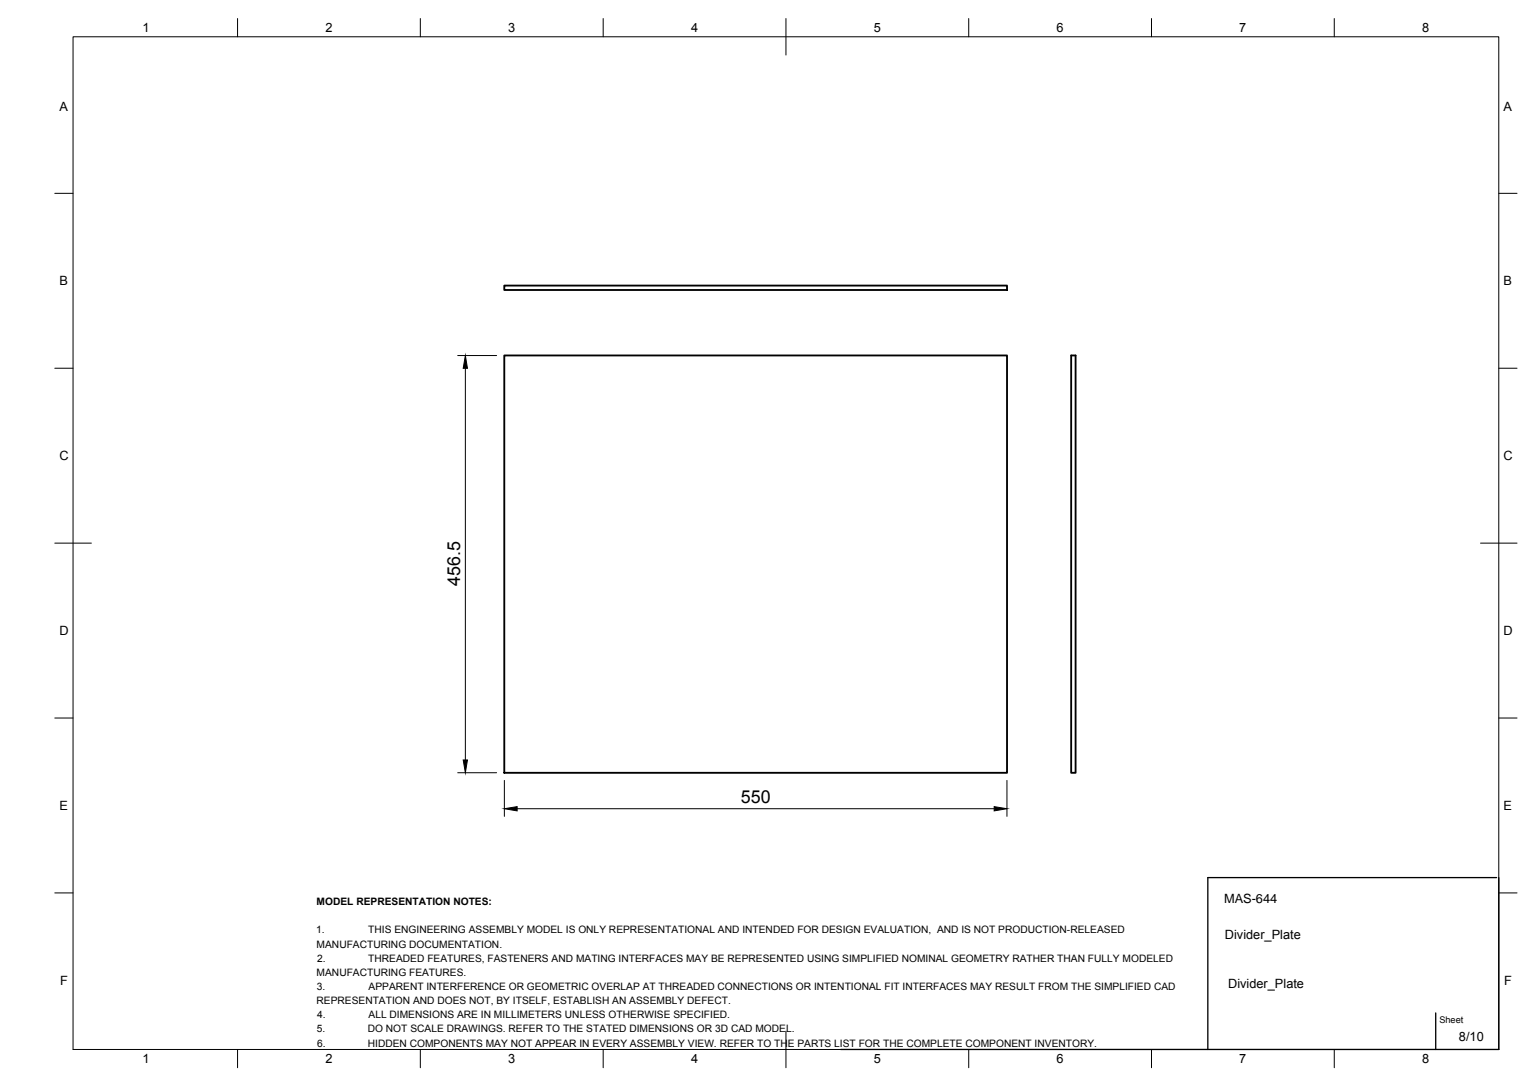
ISO-10303-21;
HEADER;
FILE_DESCRIPTION((''),'2;1');
FILE_NAME('Divider_Plate.step','2026-10-09T11:38:21-07:00',(''),(''),'','','');
FILE_SCHEMA (('AUTOMOTIVE_DESIGN { 1 0 10303 214 3 1 1 }'));
ENDSEC;
DATA;
#10=MECHANICAL_DESIGN_GEOMETRIC_PRESENTATION_REPRESENTATION('',(#64),#3619);
#48=SHAPE_REPRESENTATION_RELATIONSHIP('SRR','None',#3656,#56) ;
#56=ADVANCED_BREP_SHAPE_REPRESENTATION('',(#72),#3616) ;
#64=STYLED_ITEM('',(#3700),#72) ;
#72=MANIFOLD_SOLID_BREP('Body1',#2088) ;
#191=PLANE('',#2365) ;
#192=PLANE('',#2366) ;
#193=PLANE('',#2367) ;
#194=PLANE('',#2368) ;
#195=PLANE('',#2369) ;
#196=PLANE('',#2370) ;
#295=FACE_OUTER_BOUND('',#485,.T.) ;
#296=FACE_OUTER_BOUND('',#486,.T.) ;
#297=FACE_OUTER_BOUND('',#487,.T.) ;
#298=FACE_OUTER_BOUND('',#488,.T.) ;
#299=FACE_OUTER_BOUND('',#489,.T.) ;
#300=FACE_OUTER_BOUND('',#490,.T.) ;
#485=EDGE_LOOP('',(#1819,#1820,#1821,#1822)) ;
#486=EDGE_LOOP('',(#1823,#1824,#1825,#1826)) ;
#487=EDGE_LOOP('',(#1827,#1828,#1829,#1830)) ;
#488=EDGE_LOOP('',(#1831,#1832,#1833,#1834)) ;
#489=EDGE_LOOP('',(#1835,#1836,#1837,#1838)) ;
#490=EDGE_LOOP('',(#1839,#1840,#1841,#1842)) ;
#631=LINE('',#3483,#795) ;
#632=LINE('',#3485,#796) ;
#633=LINE('',#3487,#797) ;
#634=LINE('',#3488,#798) ;
#635=LINE('',#3491,#799) ;
#636=LINE('',#3493,#800) ;
#637=LINE('',#3494,#801) ;
#638=LINE('',#3497,#802) ;
#639=LINE('',#3499,#803) ;
#640=LINE('',#3500,#804) ;
#641=LINE('',#3502,#805) ;
#642=LINE('',#3503,#806) ;
#795=VECTOR('',#2901,1000.) ;
#796=VECTOR('',#2902,1000.) ;
#797=VECTOR('',#2903,1000.) ;
#798=VECTOR('',#2904,1000.) ;
#799=VECTOR('',#2907,1000.) ;
#800=VECTOR('',#2908,1000.) ;
#801=VECTOR('',#2909,1000.) ;
#802=VECTOR('',#2912,1000.) ;
#803=VECTOR('',#2913,1000.) ;
#804=VECTOR('',#2914,1000.) ;
#805=VECTOR('',#2917,1000.) ;
#806=VECTOR('',#2918,1000.) ;
#1087=VERTEX_POINT('',#3481) ;
#1088=VERTEX_POINT('',#3482) ;
#1089=VERTEX_POINT('',#3484) ;
#1090=VERTEX_POINT('',#3486) ;
#1091=VERTEX_POINT('',#3490) ;
#1092=VERTEX_POINT('',#3492) ;
#1093=VERTEX_POINT('',#3496) ;
#1094=VERTEX_POINT('',#3498) ;
#1335=EDGE_CURVE('',#1087,#1088,#631,.T.) ;
#1336=EDGE_CURVE('',#1089,#1087,#632,.T.) ;
#1337=EDGE_CURVE('',#1089,#1090,#633,.T.) ;
#1338=EDGE_CURVE('',#1090,#1088,#634,.T.) ;
#1339=EDGE_CURVE('',#1091,#1087,#635,.T.) ;
#1340=EDGE_CURVE('',#1092,#1091,#636,.T.) ;
#1341=EDGE_CURVE('',#1092,#1089,#637,.T.) ;
#1342=EDGE_CURVE('',#1093,#1091,#638,.T.) ;
#1343=EDGE_CURVE('',#1094,#1093,#639,.T.) ;
#1344=EDGE_CURVE('',#1094,#1092,#640,.T.) ;
#1345=EDGE_CURVE('',#1088,#1093,#641,.T.) ;
#1346=EDGE_CURVE('',#1090,#1094,#642,.T.) ;
#1819=ORIENTED_EDGE('',*,*,#1335,.F.) ;
#1820=ORIENTED_EDGE('',*,*,#1336,.F.) ;
#1821=ORIENTED_EDGE('',*,*,#1337,.T.) ;
#1822=ORIENTED_EDGE('',*,*,#1338,.T.) ;
#1823=ORIENTED_EDGE('',*,*,#1339,.F.) ;
#1824=ORIENTED_EDGE('',*,*,#1340,.F.) ;
#1825=ORIENTED_EDGE('',*,*,#1341,.T.) ;
#1826=ORIENTED_EDGE('',*,*,#1336,.T.) ;
#1827=ORIENTED_EDGE('',*,*,#1342,.F.) ;
#1828=ORIENTED_EDGE('',*,*,#1343,.F.) ;
#1829=ORIENTED_EDGE('',*,*,#1344,.T.) ;
#1830=ORIENTED_EDGE('',*,*,#1340,.T.) ;
#1831=ORIENTED_EDGE('',*,*,#1345,.F.) ;
#1832=ORIENTED_EDGE('',*,*,#1338,.F.) ;
#1833=ORIENTED_EDGE('',*,*,#1346,.T.) ;
#1834=ORIENTED_EDGE('',*,*,#1343,.T.) ;
#1835=ORIENTED_EDGE('',*,*,#1337,.F.) ;
#1836=ORIENTED_EDGE('',*,*,#1341,.F.) ;
#1837=ORIENTED_EDGE('',*,*,#1344,.F.) ;
#1838=ORIENTED_EDGE('',*,*,#1346,.F.) ;
#1839=ORIENTED_EDGE('',*,*,#1335,.T.) ;
#1840=ORIENTED_EDGE('',*,*,#1345,.T.) ;
#1841=ORIENTED_EDGE('',*,*,#1342,.T.) ;
#1842=ORIENTED_EDGE('',*,*,#1339,.T.) ;
#2057=ADVANCED_FACE('',(#295),#191,.T.) ;
#2058=ADVANCED_FACE('',(#296),#192,.T.) ;
#2059=ADVANCED_FACE('',(#297),#193,.T.) ;
#2060=ADVANCED_FACE('',(#298),#194,.T.) ;
#2061=ADVANCED_FACE('',(#299),#195,.F.) ;
#2062=ADVANCED_FACE('',(#300),#196,.T.) ;
#2088=CLOSED_SHELL('',(#2057,#2058,#2059,#2060,#2061,#2062)) ;
#2364=AXIS2_PLACEMENT_3D('',#3479,#2897,#2898) ;
#2365=AXIS2_PLACEMENT_3D('',#3480,#2899,#2900) ;
#2366=AXIS2_PLACEMENT_3D('',#3489,#2905,#2906) ;
#2367=AXIS2_PLACEMENT_3D('',#3495,#2910,#2911) ;
#2368=AXIS2_PLACEMENT_3D('',#3501,#2915,#2916) ;
#2369=AXIS2_PLACEMENT_3D('',#3504,#2919,#2920) ;
#2370=AXIS2_PLACEMENT_3D('',#3505,#2921,#2922) ;
#2897=DIRECTION('axis',(0.,0.,1.)) ;
#2898=DIRECTION('refdir',(1.,0.,0.)) ;
#2899=DIRECTION('center_axis',(3.11423403168202E-19,-2.44394566430984E-20,
1.)) ;
#2900=DIRECTION('ref_axis',(1.,-1.80411241501588E-16,-3.11423403168202E-19)) ;
#2901=DIRECTION('',(1.80411241501588E-16,1.,2.44394566430984E-20)) ;
#2902=DIRECTION('',(-1.,1.80411241501588E-16,3.11423403168202E-19)) ;
#2903=DIRECTION('',(1.80411241501588E-16,1.,2.44394566430984E-20)) ;
#2904=DIRECTION('',(-1.,1.80411241501588E-16,3.11423403168202E-19)) ;
#2905=DIRECTION('center_axis',(-1.80411241501588E-16,-1.,-2.44394566430983E-20)) ;
#2906=DIRECTION('ref_axis',(1.,-1.80411241501588E-16,-3.11423403168202E-19)) ;
#2907=DIRECTION('',(3.11423403168202E-19,-2.44394566430984E-20,1.)) ;
#2908=DIRECTION('',(-1.,1.80411241501588E-16,3.11423403168202E-19)) ;
#2909=DIRECTION('',(3.11423403168202E-19,-2.44394566430984E-20,1.)) ;
#2910=DIRECTION('center_axis',(-3.11423403168238E-19,-2.01834292293385E-16,
-1.)) ;
#2911=DIRECTION('ref_axis',(-1.80411241501588E-16,-1.,2.01834292293385E-16)) ;
#2912=DIRECTION('',(-1.80411241501588E-16,-1.,2.01834292293385E-16)) ;
#2913=DIRECTION('',(-1.,1.80411241501588E-16,3.11423403168202E-19)) ;
#2914=DIRECTION('',(-1.80411241501588E-16,-1.,2.01834292293385E-16)) ;
#2915=DIRECTION('center_axis',(1.80411241501588E-16,1.,2.44394566430983E-20)) ;
#2916=DIRECTION('ref_axis',(-1.,1.80411241501588E-16,3.11423403168202E-19)) ;
#2917=DIRECTION('',(-3.11423403168202E-19,2.44394566430984E-20,-1.)) ;
#2918=DIRECTION('',(-3.11423403168202E-19,2.44394566430984E-20,-1.)) ;
#2919=DIRECTION('center_axis',(-1.,1.80411241501588E-16,3.11423403168202E-19)) ;
#2920=DIRECTION('ref_axis',(3.11423403168202E-19,-2.44394566430984E-20,
1.)) ;
#2921=DIRECTION('center_axis',(-1.,1.80411241501588E-16,3.11423403168202E-19)) ;
#2922=DIRECTION('ref_axis',(3.11423403168202E-19,-2.44394566430984E-20,
1.)) ;
#3479=CARTESIAN_POINT('',(0.,0.,0.)) ;
#3480=CARTESIAN_POINT('Origin',(884.999999999999,550.,456.5)) ;
#3481=CARTESIAN_POINT('',(880.239999999999,5.55111512312578E-14,456.5)) ;
#3482=CARTESIAN_POINT('',(880.239999999999,550.,456.5)) ;
#3483=CARTESIAN_POINT('',(880.239999999999,550.,456.5)) ;
#3484=CARTESIAN_POINT('',(884.999999999999,5.55111512312578E-14,456.5)) ;
#3485=CARTESIAN_POINT('',(884.999999999999,5.55111512312578E-14,456.5)) ;
#3486=CARTESIAN_POINT('',(884.999999999999,550.,456.5)) ;
#3487=CARTESIAN_POINT('',(884.999999999999,550.,456.5)) ;
#3488=CARTESIAN_POINT('',(884.999999999999,550.,456.5)) ;
#3489=CARTESIAN_POINT('Origin',(884.999999999999,5.55111512312578E-14,5.55111512312578E-14)) ;
#3490=CARTESIAN_POINT('',(880.239999999999,5.55111512312578E-14,5.55111512312578E-14)) ;
#3491=CARTESIAN_POINT('',(880.239999999999,5.55111512312578E-14,5.55111512312578E-14)) ;
#3492=CARTESIAN_POINT('',(884.999999999999,5.55111512312578E-14,5.55111512312578E-14)) ;
#3493=CARTESIAN_POINT('',(884.999999999999,5.55111512312578E-14,5.55111512312578E-14)) ;
#3494=CARTESIAN_POINT('',(884.999999999999,5.55111512312578E-14,5.55111512312578E-14)) ;
#3495=CARTESIAN_POINT('Origin',(884.999999999999,550.,-5.55111512312578E-14)) ;
#3496=CARTESIAN_POINT('',(880.239999999999,550.,-5.55111512312578E-14)) ;
#3497=CARTESIAN_POINT('',(880.239999999999,550.,-5.55111512312578E-14)) ;
#3498=CARTESIAN_POINT('',(884.999999999999,550.,-5.55111512312578E-14)) ;
#3499=CARTESIAN_POINT('',(884.999999999999,550.,-5.55111512312578E-14)) ;
#3500=CARTESIAN_POINT('',(884.999999999999,550.,-5.55111512312578E-14)) ;
#3501=CARTESIAN_POINT('Origin',(884.999999999999,550.,-5.55111512312578E-14)) ;
#3502=CARTESIAN_POINT('',(880.239999999999,550.,-5.55111512312578E-14)) ;
#3503=CARTESIAN_POINT('',(884.999999999999,550.,-5.55111512312578E-14)) ;
#3504=CARTESIAN_POINT('Origin',(884.999999999999,275.,228.25)) ;
#3505=CARTESIAN_POINT('Origin',(880.239999999999,275.,228.25)) ;
#3606=UNCERTAINTY_MEASURE_WITH_UNIT(LENGTH_MEASURE(0.01),#3620,
'DISTANCE_ACCURACY_VALUE',
'Maximum model space distance between geometric entities at asserted c
onnectivities') ;
#3609=UNCERTAINTY_MEASURE_WITH_UNIT(LENGTH_MEASURE(0.01),#3620,
'DISTANCE_ACCURACY_VALUE',
'Maximum model space distance between geometric entities at asserted c
onnectivities') ;
#3616=(
GEOMETRIC_REPRESENTATION_CONTEXT(3)
GLOBAL_UNCERTAINTY_ASSIGNED_CONTEXT((#3606))
GLOBAL_UNIT_ASSIGNED_CONTEXT((#3620,#3622,#3623))
REPRESENTATION_CONTEXT('','3D')
) ;
#3619=(
GEOMETRIC_REPRESENTATION_CONTEXT(3)
GLOBAL_UNCERTAINTY_ASSIGNED_CONTEXT((#3609))
GLOBAL_UNIT_ASSIGNED_CONTEXT((#3620,#3622,#3623))
REPRESENTATION_CONTEXT('','3D')
) ;
#3620=(
LENGTH_UNIT()
NAMED_UNIT(*)
SI_UNIT(.MILLI.,.METRE.)
) ;
#3622=(
NAMED_UNIT(*)
PLANE_ANGLE_UNIT()
SI_UNIT($,.RADIAN.)
) ;
#3623=(
NAMED_UNIT(*)
SI_UNIT($,.STERADIAN.)
SOLID_ANGLE_UNIT()
) ;
#3630=SHAPE_DEFINITION_REPRESENTATION(#3639,#3656) ;
#3639=PRODUCT_DEFINITION_SHAPE('',$,#3666) ;
#3656=SHAPE_REPRESENTATION('',(#2364),#3616) ;
#3659=PRODUCT_DEFINITION_CONTEXT('part definition',#3688,'design') ;
#3666=PRODUCT_DEFINITION('Divider_Plate','Divider_Plate',#3675,#3659) ;
#3675=PRODUCT_DEFINITION_FORMATION('',$,#3696) ;
#3688=APPLICATION_CONTEXT(
'Core Data for Automotive Mechanical Design Process') ;
#3689=PRODUCT_CONTEXT('part definition',#3688,'mechanical') ;
#3696=PRODUCT('Divider_Plate','Divider_Plate',$,(#3689)) ;
#3700=PRESENTATION_STYLE_ASSIGNMENT((#3702)) ;
#3702=SURFACE_STYLE_USAGE(.BOTH.,#3704) ;
#3704=SURFACE_SIDE_STYLE('',(#3706)) ;
#3706=SURFACE_STYLE_FILL_AREA(#3708) ;
#3708=FILL_AREA_STYLE('Opaque(202,209,238)',(#3710)) ;
#3710=FILL_AREA_STYLE_COLOUR('Opaque(202,209,238)',#3712) ;
#3712=COLOUR_RGB('Opaque(202,209,238)', 0.09019608, 0.27058824, 0.51372549) ;
ENDSEC;
END-ISO-10303-21;
